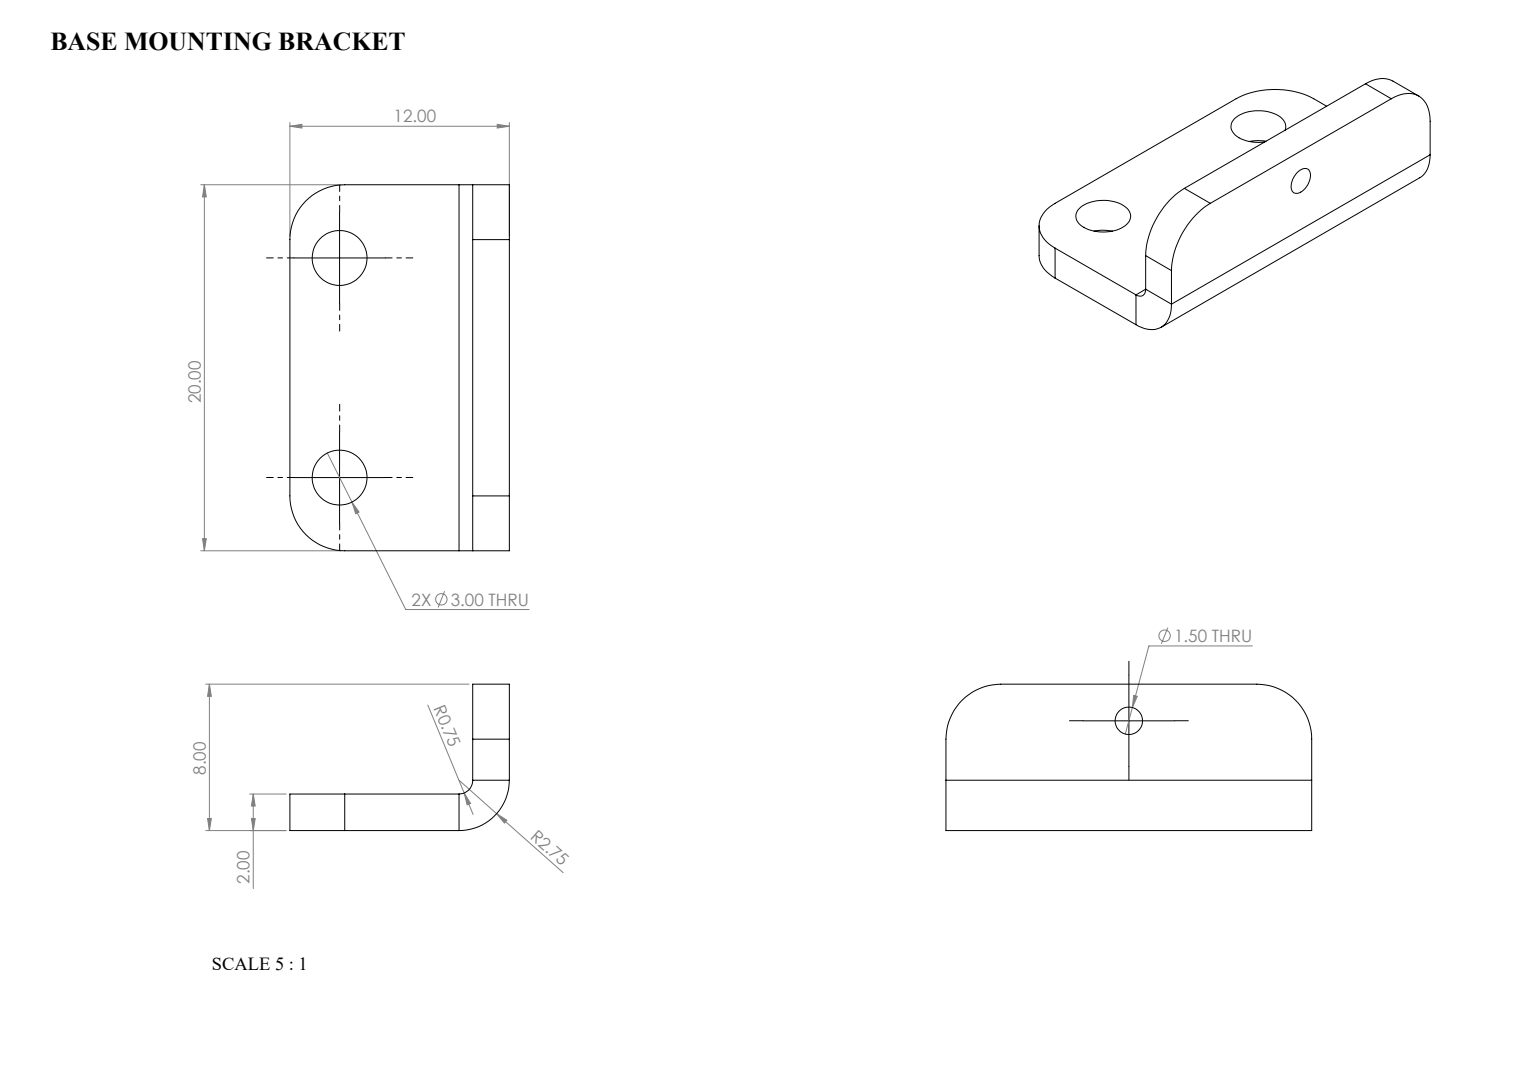
ISO-10303-21;
HEADER;
FILE_DESCRIPTION (('STEP AP214'),
    '1' );
FILE_NAME ('base-mounting-bracket.step',
    '2026-10-11T23:18:24',
    ( '' ),
    ( '' ),
    'SwSTEP 2.0',
    'SolidWorks 2021',
    '' );
FILE_SCHEMA (( 'AUTOMOTIVE_DESIGN' ));
ENDSEC;

DATA;
#8=ORIENTED_EDGE ( 'NONE', *, *, #949, .F. ) ;
#37=FACE_OUTER_BOUND ( 'NONE', #7927, .T. ) ;
#43=VERTEX_POINT ( 'NONE', #6242 ) ;
#47=FACE_BOUND ( 'NONE', #7549, .T. ) ;
#50=CIRCLE ( 'NONE', #7727, 3.000000000000000000 ) ;
#51=FACE_OUTER_BOUND ( 'NONE', #63, .T. ) ;
#63=EDGE_LOOP ( 'NONE', ( #5168, #8136, #3931, #2663 ) ) ;
#72=CARTESIAN_POINT ( 'NONE',  ( 10.00000000000000000, 2.749999999999999112, -10.00000000000000178 ) ) ;
#122=AXIS2_PLACEMENT_3D ( 'NONE', #7328, #11458, #1060 ) ;
#142=FACE_OUTER_BOUND ( 'NONE', #3099, .T. ) ;
#145=ORIENTED_EDGE ( 'NONE', *, *, #11996, .T. ) ;
#170=DIRECTION ( 'NONE',  ( -2.602085213965199795E-16, 2.891205793294684736E-16, -1.000000000000000000 ) ) ;
#212=EDGE_CURVE ( 'NONE', #8880, #8783, #12663, .T. ) ;
#240=ORIENTED_EDGE ( 'NONE', *, *, #11722, .F. ) ;
#241=DIRECTION ( 'NONE',  ( 0.000000000000000000, 1.000000000000000000, -0.000000000000000000 ) ) ;
#257=LINE ( 'NONE', #1752, #8132 ) ;
#264=EDGE_CURVE ( 'NONE', #8710, #692, #9279, .T. ) ;
#268=EDGE_LOOP ( 'NONE', ( #11853, #9948, #1249, #11697 ) ) ;
#271=EDGE_CURVE ( 'NONE', #7435, #2693, #13455, .T. ) ;
#304=DIRECTION ( 'NONE',  ( 0.000000000000000000, 1.000000000000000000, 0.000000000000000000 ) ) ;
#311=CIRCLE ( 'NONE', #11742, 3.000000000000000000 ) ;
#329=CARTESIAN_POINT ( 'NONE',  ( 2.720000000000001528, 2.000000000000000000, 7.500000000000000888 ) ) ;
#374=ORIENTED_EDGE ( 'NONE', *, *, #11346, .F. ) ;
#420=CARTESIAN_POINT ( 'NONE',  ( 2.720000000000001528, 0.000000000000000000, 4.500000000000000000 ) ) ;
#425=ORIENTED_EDGE ( 'NONE', *, *, #11861, .F. ) ;
#444=EDGE_CURVE ( 'NONE', #11209, #5642, #3242, .T. ) ;
#445=MECHANICAL_DESIGN_GEOMETRIC_PRESENTATION_REPRESENTATION('',(#6386),#6171);
#474=LINE ( 'NONE', #4679, #13306 ) ;
#486=ORIENTED_EDGE ( 'NONE', *, *, #11722, .T. ) ;
#489=( NAMED_UNIT ( * ) SI_UNIT ( $, .STERADIAN. ) SOLID_ANGLE_UNIT ( ) );
#491=AXIS2_PLACEMENT_3D ( 'NONE', #848, #12295, #6081 ) ;
#519=VECTOR ( 'NONE', #1899, 1000.000000000000000 ) ;
#559=EDGE_LOOP ( 'NONE', ( #8381, #3710, #2080, #13458 ) ) ;
#563=LINE ( 'NONE', #1798, #9730 ) ;
#590=DIRECTION ( 'NONE',  ( 0.000000000000000000, 0.000000000000000000, 1.000000000000000000 ) ) ;
#599=FACE_OUTER_BOUND ( 'NONE', #1472, .T. ) ;
#603=DIRECTION ( 'NONE',  ( 1.000000000000000000, -3.469446951953610639E-15, -2.602085213965210149E-16 ) ) ;
#608=ORIENTED_EDGE ( 'NONE', *, *, #6998, .F. ) ;
#614=ADVANCED_FACE ( 'NONE', ( #3441 ), #10691, .F. ) ;
#631=DIRECTION ( 'NONE',  ( 0.000000000000000000, 0.000000000000000000, -1.000000000000000000 ) ) ;
#639=ADVANCED_BREP_SHAPE_REPRESENTATION ( '', ( #3911, #10007 ), #12660 ) ;
#648=DIRECTION ( 'NONE',  ( -3.469446951953614189E-15, -1.000000000000000000, 8.673617379884035472E-16 ) ) ;
#687=LINE ( 'NONE', #5850, #12010 ) ;
#692=VERTEX_POINT ( 'NONE', #11854 ) ;
#697=ORIENTED_EDGE ( 'NONE', *, *, #1747, .T. ) ;
#707=EDGE_CURVE ( 'NONE', #8736, #9662, #5546, .T. ) ;
#736=EDGE_CURVE ( 'NONE', #7676, #11515, #12131, .T. ) ;
#740=AXIS2_PLACEMENT_3D ( 'NONE', #5209, #10447, #871 ) ;
#808=ORIENTED_EDGE ( 'NONE', *, *, #12116, .F. ) ;
#810=LINE ( 'NONE', #12316, #2307 ) ;
#848=CARTESIAN_POINT ( 'NONE',  ( 10.00000000000001421, 6.000000000000007105, -2.602085213965208275E-15 ) ) ;
#854=DIRECTION ( 'NONE',  ( -1.000000000000000000, 0.000000000000000000, -0.000000000000000000 ) ) ;
#865=ORIENTED_EDGE ( 'NONE', *, *, #444, .T. ) ;
#871=DIRECTION ( 'NONE',  ( 0.000000000000000000, 0.000000000000000000, 1.000000000000000000 ) ) ;
#872=EDGE_CURVE ( 'NONE', #8783, #8207, #563, .T. ) ;
#901=SURFACE_SIDE_STYLE ('',( #11166 ) ) ;
#940=LINE ( 'NONE', #9342, #5056 ) ;
#949=EDGE_CURVE ( 'NONE', #11231, #5642, #6128, .T. ) ;
#954=DIRECTION ( 'NONE',  ( 0.000000000000000000, 0.000000000000000000, 1.000000000000000000 ) ) ;
#971=DIRECTION ( 'NONE',  ( 0.000000000000000000, 0.000000000000000000, 1.000000000000000000 ) ) ;
#978=ORIENTED_EDGE ( 'NONE', *, *, #10739, .T. ) ;
#994=CARTESIAN_POINT ( 'NONE',  ( 12.00000000000000533, 2.749999999999991118, 10.00000000000000000 ) ) ;
#1001=ORIENTED_EDGE ( 'NONE', *, *, #5458, .F. ) ;
#1060=DIRECTION ( 'NONE',  ( 0.000000000000000000, 0.000000000000000000, 1.000000000000000000 ) ) ;
#1071=DIRECTION ( 'NONE',  ( -2.312964634635743450E-15, -1.000000000000000000, 0.000000000000000000 ) ) ;
#1102=EDGE_CURVE ( 'NONE', #43, #2399, #1440, .T. ) ;
#1136=DIRECTION ( 'NONE',  ( 2.602085213965210149E-16, 0.000000000000000000, 1.000000000000000000 ) ) ;
#1141=DIRECTION ( 'NONE',  ( 0.000000000000000000, 0.000000000000000000, 1.000000000000000000 ) ) ;
#1145=CIRCLE ( 'NONE', #4886, 0.7500000000000024425 ) ;
#1146=CARTESIAN_POINT ( 'NONE',  ( 3.000000000000001776, 2.000000000000000000, 10.00000000000000000 ) ) ;
#1174=CIRCLE ( 'NONE', #740, 1.499999999999999556 ) ;
#1185=ORIENTED_EDGE ( 'NONE', *, *, #10601, .F. ) ;
#1223=CARTESIAN_POINT ( 'NONE',  ( -2.551540321038929007E-15, 0.000000000000000000, -7.000000000000000000 ) ) ;
#1249=ORIENTED_EDGE ( 'NONE', *, *, #3731, .T. ) ;
#1266=VERTEX_POINT ( 'NONE', #11146 ) ;
#1282=ADVANCED_FACE ( 'NONE', ( #1650 ), #6793, .F. ) ;
#1358=EDGE_LOOP ( 'NONE', ( #6259, #10717, #6942, #8787 ) ) ;
#1361=ORIENTED_EDGE ( 'NONE', *, *, #4222, .F. ) ;
#1367=VECTOR ( 'NONE', #2475, 1000.000000000000000 ) ;
#1378=ORIENTED_EDGE ( 'NONE', *, *, #7513, .T. ) ;
#1384=DIRECTION ( 'NONE',  ( 0.000000000000000000, 1.000000000000000000, 0.000000000000000000 ) ) ;
#1395=AXIS2_PLACEMENT_3D ( 'NONE', #11099, #6753, #631 ) ;
#1399=ORIENTED_EDGE ( 'NONE', *, *, #4811, .F. ) ;
#1421=CARTESIAN_POINT ( 'NONE',  ( 9.250000000000001776, 1.999999999999998224, -10.00000000000000178 ) ) ;
#1440=LINE ( 'NONE', #9630, #11953 ) ;
#1459=DIRECTION ( 'NONE',  ( 2.602085213965199795E-16, -2.891205793294684736E-16, 1.000000000000000000 ) ) ;
#1472=EDGE_LOOP ( 'NONE', ( #7725, #6948, #2931, #9761 ) ) ;
#1499=ORIENTED_EDGE ( 'NONE', *, *, #9261, .F. ) ;
#1519=ADVANCED_FACE ( 'NONE', ( #13186 ), #3739, .T. ) ;
#1545=DIRECTION ( 'NONE',  ( 1.000000000000000000, -3.469446951953610639E-15, -2.602085213965210149E-16 ) ) ;
#1586=UNCERTAINTY_MEASURE_WITH_UNIT (LENGTH_MEASURE( 1.000000000000000082E-05 ), #6895, 'distance_accuracy_value', 'NONE');
#1610=ORIENTED_EDGE ( 'NONE', *, *, #1879, .T. ) ;
#1621=CARTESIAN_POINT ( 'NONE',  ( 20.00000000000001421, 5.999999999999972466, -5.204170427930418128E-15 ) ) ;
#1650=FACE_OUTER_BOUND ( 'NONE', #4981, .T. ) ;
#1662=VERTEX_POINT ( 'NONE', #329 ) ;
#1669=CYLINDRICAL_SURFACE ( 'NONE', #1395, 1.500000000000000444 ) ;
#1674=DIRECTION ( 'NONE',  ( -2.312964634635743450E-15, -1.000000000000000000, 0.000000000000000000 ) ) ;
#1697=ORIENTED_EDGE ( 'NONE', *, *, #10199, .F. ) ;
#1723=CARTESIAN_POINT ( 'NONE',  ( 12.00000000000001243, 4.999999999999999112, 10.00000000000000178 ) ) ;
#1732=ADVANCED_FACE ( 'NONE', ( #9746 ), #6375, .F. ) ;
#1740=CARTESIAN_POINT ( 'NONE',  ( 12.00000000000001421, 6.000000000000000000, -3.122502256758250009E-15 ) ) ;
#1747=EDGE_CURVE ( 'NONE', #2399, #7044, #7623, .T. ) ;
#1752=CARTESIAN_POINT ( 'NONE',  ( 11.99999999999999112, -4.572512030783488065E-14, -10.00000000000000178 ) ) ;
#1798=CARTESIAN_POINT ( 'NONE',  ( 3.000000000000001776, 0.000000000000000000, 10.00000000000000000 ) ) ;
#1809=LINE ( 'NONE', #6824, #4723 ) ;
#1862=LINE ( 'NONE', #7167, #5318 ) ;
#1872=ORIENTED_EDGE ( 'NONE', *, *, #3526, .F. ) ;
#1879=EDGE_CURVE ( 'NONE', #2097, #9662, #3747, .T. ) ;
#1888=EDGE_LOOP ( 'NONE', ( #6480, #9877 ) ) ;
#1899=DIRECTION ( 'NONE',  ( 1.000000000000000000, -3.491481338843133355E-15, -2.602085213965210149E-16 ) ) ;
#1913=DIRECTION ( 'NONE',  ( -0.000000000000000000, -1.000000000000000000, -0.000000000000000000 ) ) ;
#1938=FILL_AREA_STYLE_COLOUR ( '', #13317 ) ;
#1950=CARTESIAN_POINT ( 'NONE',  ( 11.99999999999999467, -5.150753189442425446E-14, 10.00000000000000000 ) ) ;
#1951=ORIENTED_EDGE ( 'NONE', *, *, #8465, .F. ) ;
#1964=EDGE_CURVE ( 'NONE', #5535, #13368, #9406, .T. ) ;
#1994=CARTESIAN_POINT ( 'NONE',  ( 2.720000000000001528, 0.000000000000000000, 7.500000000000000888 ) ) ;
#2028=DIRECTION ( 'NONE',  ( -1.000000000000000000, 3.469446951953610639E-15, 2.602085213965210149E-16 ) ) ;
#2080=ORIENTED_EDGE ( 'NONE', *, *, #1964, .F. ) ;
#2092=AXIS2_PLACEMENT_3D ( 'NONE', #6235, #2858, #3957 ) ;
#2094=CIRCLE ( 'NONE', #122, 1.500000000000000444 ) ;
#2097=VERTEX_POINT ( 'NONE', #6037 ) ;
#2109=DIRECTION ( 'NONE',  ( -3.469446951953614189E-15, -1.000000000000000000, 0.000000000000000000 ) ) ;
#2133=EDGE_CURVE ( 'NONE', #13368, #2399, #8219, .T. ) ;
#2140=LINE ( 'NONE', #5238, #4952 ) ;
#2156=DIRECTION ( 'NONE',  ( 0.000000000000000000, 1.000000000000000000, 0.000000000000000000 ) ) ;
#2165=ORIENTED_EDGE ( 'NONE', *, *, #11291, .T. ) ;
#2185=DIRECTION ( 'NONE',  ( -1.000000000000000000, 3.469446951953610639E-15, 2.602085213965210149E-16 ) ) ;
#2204=ADVANCED_FACE ( 'NONE', ( #11813, #47, #9465 ), #11610, .F. ) ;
#2231=EDGE_CURVE ( 'NONE', #9010, #7333, #4707, .T. ) ;
#2250=DIRECTION ( 'NONE',  ( -3.469446951953610639E-15, -1.000000000000000000, 0.000000000000000000 ) ) ;
#2275=ORIENTED_EDGE ( 'NONE', *, *, #8478, .T. ) ;
#2287=ADVANCED_FACE ( 'NONE', ( #11115 ), #5732, .F. ) ;
#2307=VECTOR ( 'NONE', #11268, 1000.000000000000000 ) ;
#2326=DIRECTION ( 'NONE',  ( 0.000000000000000000, 0.000000000000000000, -1.000000000000000000 ) ) ;
#2327=DIRECTION ( 'NONE',  ( 3.469446951953610639E-15, 1.000000000000000000, 2.891205793294675861E-16 ) ) ;
#2344=CARTESIAN_POINT ( 'NONE',  ( 10.00000000000002309, 8.000000000000007105, 7.000000000000001776 ) ) ;
#2365=ADVANCED_FACE ( 'NONE', ( #7127, #10285, #8279 ), #4084, .T. ) ;
#2394=ORIENTED_EDGE ( 'NONE', *, *, #444, .F. ) ;
#2399=VERTEX_POINT ( 'NONE', #10346 ) ;
#2475=DIRECTION ( 'NONE',  ( -1.000000000000000000, 3.491481338843133355E-15, 2.602085213965210149E-16 ) ) ;
#2485=ORIENTED_EDGE ( 'NONE', *, *, #264, .T. ) ;
#2508=CARTESIAN_POINT ( 'NONE',  ( 12.00000000000000888, 5.000000000000000000, -6.999999999999999112 ) ) ;
#2573=DIRECTION ( 'NONE',  ( -0.000000000000000000, -1.000000000000000000, -0.000000000000000000 ) ) ;
#2621=ADVANCED_FACE ( 'NONE', ( #9786 ), #1669, .F. ) ;
#2627=ORIENTED_EDGE ( 'NONE', *, *, #10538, .T. ) ;
#2658=CARTESIAN_POINT ( 'NONE',  ( 3.000000000000001776, 2.000000000000000000, 10.00000000000000000 ) ) ;
#2663=ORIENTED_EDGE ( 'NONE', *, *, #271, .F. ) ;
#2686=( NAMED_UNIT ( * ) SI_UNIT ( $, .STERADIAN. ) SOLID_ANGLE_UNIT ( ) );
#2693=VERTEX_POINT ( 'NONE', #12900 ) ;
#2695=ADVANCED_FACE ( 'NONE', ( #8882 ), #3711, .T. ) ;
#2702=AXIS2_PLACEMENT_3D ( 'NONE', #12467, #3258, #1071 ) ;
#2735=CARTESIAN_POINT ( 'NONE',  ( 10.00000000000001243, 5.000000000000007105, 7.000000000000001776 ) ) ;
#2761=ORIENTED_EDGE ( 'NONE', *, *, #949, .T. ) ;
#2825=EDGE_CURVE ( 'NONE', #5427, #12707, #3934, .T. ) ;
#2847=DIRECTION ( 'NONE',  ( 0.000000000000000000, 1.000000000000000000, 0.000000000000000000 ) ) ;
#2858=DIRECTION ( 'NONE',  ( -0.000000000000000000, -0.000000000000000000, -1.000000000000000000 ) ) ;
#2867=EDGE_CURVE ( 'NONE', #12707, #5427, #12317, .T. ) ;
#2879=DIRECTION ( 'NONE',  ( -1.000000000000000000, 3.469446951953610639E-15, 2.602085213965210149E-16 ) ) ;
#2895=FILL_AREA_STYLE ('',( #1938 ) ) ;
#2896=CARTESIAN_POINT ( 'NONE',  ( 12.00000000000002309, 8.000000000000000000, 7.000000000000000888 ) ) ;
#2929=ORIENTED_EDGE ( 'NONE', *, *, #11861, .T. ) ;
#2931=ORIENTED_EDGE ( 'NONE', *, *, #8943, .F. ) ;
#2947=EDGE_LOOP ( 'NONE', ( #11195, #11654, #6079, #11465 ) ) ;
#2956=PLANE ( 'NONE',  #12210 ) ;
#2957=VECTOR ( 'NONE', #2879, 1000.000000000000000 ) ;
#3056=AXIS2_PLACEMENT_3D ( 'NONE', #10125, #12284, #971 ) ;
#3083=DIRECTION ( 'NONE',  ( -1.000000000000000000, -0.000000000000000000, -1.927470528863118802E-16 ) ) ;
#3099=EDGE_LOOP ( 'NONE', ( #12485, #7712, #865, #8, #13124, #4158 ) ) ;
#3149=FACE_BOUND ( 'NONE', #3474, .T. ) ;
#3184=CARTESIAN_POINT ( 'NONE',  ( 2.719999999999997087, 2.000000000000000000, -6.000000000000000000 ) ) ;
#3191=PLANE ( 'NONE',  #6195 ) ;
#3202=DIRECTION ( 'NONE',  ( 0.000000000000000000, -0.000000000000000000, 1.000000000000000000 ) ) ;
#3204=DIRECTION ( 'NONE',  ( 1.000000000000000000, 0.000000000000000000, -0.000000000000000000 ) ) ;
#3242=LINE ( 'NONE', #1950, #11944 ) ;
#3251=ORIENTED_EDGE ( 'NONE', *, *, #872, .T. ) ;
#3258=DIRECTION ( 'NONE',  ( -1.000000000000000000, 3.469446951953610639E-15, 2.602085213965210149E-16 ) ) ;
#3266=ORIENTED_EDGE ( 'NONE', *, *, #4811, .T. ) ;
#3381=DIRECTION ( 'NONE',  ( 0.000000000000000000, 0.000000000000000000, 1.000000000000000000 ) ) ;
#3435=CARTESIAN_POINT ( 'NONE',  ( 2.999999999999997335, 2.000000000000000000, -7.000000000000001776 ) ) ;
#3441=FACE_OUTER_BOUND ( 'NONE', #4881, .T. ) ;
#3460=EDGE_CURVE ( 'NONE', #9662, #8736, #4395, .T. ) ;
#3465=DIRECTION ( 'NONE',  ( 1.000000000000000000, -3.469446951953610639E-15, 0.000000000000000000 ) ) ;
#3474=EDGE_LOOP ( 'NONE', ( #978, #8024 ) ) ;
#3486=EDGE_LOOP ( 'NONE', ( #1951, #2929, #1610, #4440 ) ) ;
#3504=CARTESIAN_POINT ( 'NONE',  ( 12.00000000000001776, 8.000000000000000000, -10.00000000000000000 ) ) ;
#3506=ORIENTED_EDGE ( 'NONE', *, *, #707, .T. ) ;
#3508=CIRCLE ( 'NONE', #10568, 1.499999999999999556 ) ;
#3526=EDGE_CURVE ( 'NONE', #11231, #9693, #257, .T. ) ;
#3537=ORIENTED_EDGE ( 'NONE', *, *, #736, .T. ) ;
#3582=DIRECTION ( 'NONE',  ( -1.000000000000000000, 3.491481338843133355E-15, 2.602085213965210149E-16 ) ) ;
#3645=UNCERTAINTY_MEASURE_WITH_UNIT (LENGTH_MEASURE( 1.000000000000000082E-05 ), #12139, 'distance_accuracy_value', 'NONE');
#3706=ORIENTED_EDGE ( 'NONE', *, *, #8465, .T. ) ;
#3710=ORIENTED_EDGE ( 'NONE', *, *, #5809, .T. ) ;
#3711=CYLINDRICAL_SURFACE ( 'NONE', #7428, 3.000000000000000000 ) ;
#3727=VECTOR ( 'NONE', #13392, 1000.000000000000000 ) ;
#3731=EDGE_CURVE ( 'NONE', #6099, #8207, #4986, .T. ) ;
#3739=PLANE ( 'NONE',  #6891 ) ;
#3747=LINE ( 'NONE', #13269, #5349 ) ;
#3809=ADVANCED_FACE ( 'NONE', ( #9653 ), #7656, .F. ) ;
#3814=CARTESIAN_POINT ( 'NONE',  ( 2.719999999999997087, 2.000000000000000000, -6.000000000000000000 ) ) ;
#3817=AXIS2_PLACEMENT_3D ( 'NONE', #10664, #10589, #2326 ) ;
#3866=DIRECTION ( 'NONE',  ( -0.000000000000000000, -0.000000000000000000, -1.000000000000000000 ) ) ;
#3880=CARTESIAN_POINT ( 'NONE',  ( 10.00000000000000533, 2.749999999999997335, 10.00000000000000178 ) ) ;
#3911=MANIFOLD_SOLID_BREP ( 'Fillet1', #5975 ) ;
#3925=DIRECTION ( 'NONE',  ( -4.625929269271486900E-15, -1.000000000000000000, 0.000000000000000000 ) ) ;
#3931=ORIENTED_EDGE ( 'NONE', *, *, #13097, .T. ) ;
#3934=CIRCLE ( 'NONE', #3056, 1.499999999999999556 ) ;
#3935=ORIENTED_EDGE ( 'NONE', *, *, #7589, .T. ) ;
#3957=DIRECTION ( 'NONE',  ( -1.000000000000000000, 0.000000000000000000, 0.000000000000000000 ) ) ;
#3984=CARTESIAN_POINT ( 'NONE',  ( 2.999999999999995559, 2.000000000000000000, -10.00000000000000355 ) ) ;
#4040=ADVANCED_FACE ( 'NONE', ( #13378 ), #10272, .F. ) ;
#4052=DIRECTION ( 'NONE',  ( -1.927470528863118802E-16, 0.000000000000000000, 1.000000000000000000 ) ) ;
#4069=CARTESIAN_POINT ( 'NONE',  ( 12.00000000000001599, 6.750000000000000000, -2.770445225425678373E-15 ) ) ;
#4084=PLANE ( 'NONE',  #8441 ) ;
#4099=ORIENTED_EDGE ( 'NONE', *, *, #5220, .T. ) ;
#4158=ORIENTED_EDGE ( 'NONE', *, *, #5458, .T. ) ;
#4168=ORIENTED_EDGE ( 'NONE', *, *, #11566, .F. ) ;
#4196=DIRECTION ( 'NONE',  ( 0.000000000000000000, 0.000000000000000000, -1.000000000000000000 ) ) ;
#4222=EDGE_CURVE ( 'NONE', #8880, #6099, #8464, .T. ) ;
#4230=CARTESIAN_POINT ( 'NONE',  ( 3.000000000000001776, 0.000000000000000000, 7.000000000000000000 ) ) ;
#4232=PLANE ( 'NONE',  #4692 ) ;
#4246=PRODUCT_DEFINITION_SHAPE ( 'NONE', 'NONE',  #5460 ) ;
#4273=DIRECTION ( 'NONE',  ( 1.000000000000000000, -3.469446951953602750E-15, 0.000000000000000000 ) ) ;
#4302=CIRCLE ( 'NONE', #10463, 3.000000000000000000 ) ;
#4317=VERTEX_POINT ( 'NONE', #6875 ) ;
#4331=ORIENTED_EDGE ( 'NONE', *, *, #10538, .F. ) ;
#4375=ORIENTED_EDGE ( 'NONE', *, *, #13136, .T. ) ;
#4390=VERTEX_POINT ( 'NONE', #12196 ) ;
#4395=CIRCLE ( 'NONE', #12763, 1.500000000000000444 ) ;
#4404=APPLICATION_CONTEXT ( 'automotive_design' ) ;
#4417=DIRECTION ( 'NONE',  ( -0.000000000000000000, -1.000000000000000000, -0.000000000000000000 ) ) ;
#4439=CARTESIAN_POINT ( 'NONE',  ( 10.00000000000001243, 5.000000000000006217, 10.00000000000000178 ) ) ;
#4440=ORIENTED_EDGE ( 'NONE', *, *, #707, .F. ) ;
#4534=ORIENTED_EDGE ( 'NONE', *, *, #3731, .F. ) ;
#4535=DIRECTION ( 'NONE',  ( -0.000000000000000000, -1.000000000000000000, -0.000000000000000000 ) ) ;
#4545=CYLINDRICAL_SURFACE ( 'NONE', #7126, 3.000000000000000000 ) ;
#4585=ORIENTED_EDGE ( 'NONE', *, *, #13097, .F. ) ;
#4617=AXIS2_PLACEMENT_3D ( 'NONE', #1621, #5816, #10014 ) ;
#4633=DIRECTION ( 'NONE',  ( 2.602085213965210149E-16, -0.000000000000000000, 1.000000000000000000 ) ) ;
#4657=VECTOR ( 'NONE', #5345, 1000.000000000000000 ) ;
#4679=CARTESIAN_POINT ( 'NONE',  ( 12.00000000000000355, 2.749999999999990230, 10.00000000000000000 ) ) ;
#4692=AXIS2_PLACEMENT_3D ( 'NONE', #8428, #12653, #3204 ) ;
#4703=AXIS2_PLACEMENT_3D ( 'NONE', #7037, #6758, #1674 ) ;
#4707=LINE ( 'NONE', #4778, #10156 ) ;
#4723=VECTOR ( 'NONE', #4771, 1000.000000000000000 ) ;
#4771=DIRECTION ( 'NONE',  ( -0.000000000000000000, -1.000000000000000000, -0.000000000000000000 ) ) ;
#4778=CARTESIAN_POINT ( 'NONE',  ( 10.00000000000002309, 8.000000000000007105, 10.00000000000000178 ) ) ;
#4782=CARTESIAN_POINT ( 'NONE',  ( 2.719999999999997087, 0.000000000000000000, -4.500000000000000888 ) ) ;
#4787=DIRECTION ( 'NONE',  ( 0.000000000000000000, 1.000000000000000000, -0.000000000000000000 ) ) ;
#4793=DIRECTION ( 'NONE',  ( -3.469446951953614189E-15, -1.000000000000000000, 0.000000000000000000 ) ) ;
#4811=EDGE_CURVE ( 'NONE', #9688, #692, #4936, .T. ) ;
#4845=FACE_OUTER_BOUND ( 'NONE', #7120, .T. ) ;
#4881=EDGE_LOOP ( 'NONE', ( #8205, #2627, #1872, #4168 ) ) ;
#4886=AXIS2_PLACEMENT_3D ( 'NONE', #7738, #10917, #11752 ) ;
#4894=CARTESIAN_POINT ( 'NONE',  ( 20.00000000000001421, 5.999999999999972466, -5.204170427930418128E-15 ) ) ;
#4895=AXIS2_PLACEMENT_3D ( 'NONE', #3504, #1459, #9910 ) ;
#4902=CYLINDRICAL_SURFACE ( 'NONE', #11110, 0.7500000000000024425 ) ;
#4910=VECTOR ( 'NONE', #6198, 1000.000000000000000 ) ;
#4936=LINE ( 'NONE', #9055, #10113 ) ;
#4952=VECTOR ( 'NONE', #13448, 1000.000000000000000 ) ;
#4959=CARTESIAN_POINT ( 'NONE',  ( 10.00000000000001243, 5.250000000000007105, -2.602085213965208275E-15 ) ) ;
#4981=EDGE_LOOP ( 'NONE', ( #697, #12186, #7245, #12343 ) ) ;
#4986=LINE ( 'NONE', #9179, #3727 ) ;
#4989=LINE ( 'NONE', #3880, #13457 ) ;
#5020=LINE ( 'NONE', #3984, #6939 ) ;
#5031=EDGE_CURVE ( 'NONE', #4317, #12707, #940, .T. ) ;
#5032=DIRECTION ( 'NONE',  ( -0.000000000000000000, -1.000000000000000000, -0.000000000000000000 ) ) ;
#5056=VECTOR ( 'NONE', #8300, 1000.000000000000000 ) ;
#5057=AXIS2_PLACEMENT_3D ( 'NONE', #9448, #170, #12834 ) ;
#5058=ORIENTED_EDGE ( 'NONE', *, *, #872, .F. ) ;
#5085=CARTESIAN_POINT ( 'NONE',  ( 20.00000000000001066, 5.249999999999972466, -5.204170427930418128E-15 ) ) ;
#5091=ORIENTED_EDGE ( 'NONE', *, *, #12432, .F. ) ;
#5131=ADVANCED_FACE ( 'NONE', ( #9809 ), #9669, .T. ) ;
#5168=ORIENTED_EDGE ( 'NONE', *, *, #7731, .F. ) ;
#5170=CIRCLE ( 'NONE', #7155, 1.500000000000000444 ) ;
#5209=CARTESIAN_POINT ( 'NONE',  ( 2.719999999999997087, 2.000000000000000000, -6.000000000000000000 ) ) ;
#5220=EDGE_CURVE ( 'NONE', #11515, #1266, #4989, .T. ) ;
#5238=CARTESIAN_POINT ( 'NONE',  ( 10.00000000000001954, 8.000000000000007105, -10.00000000000000000 ) ) ;
#5292=ADVANCED_FACE ( 'NONE', ( #4845 ), #12304, .F. ) ;
#5309=EDGE_CURVE ( 'NONE', #6406, #4317, #3508, .T. ) ;
#5318=VECTOR ( 'NONE', #1141, 1000.000000000000000 ) ;
#5324=ORIENTED_EDGE ( 'NONE', *, *, #12397, .T. ) ;
#5329=AXIS2_PLACEMENT_3D ( 'NONE', #10813, #1384, #5580 ) ;
#5345=DIRECTION ( 'NONE',  ( -0.000000000000000000, -1.000000000000000000, -0.000000000000000000 ) ) ;
#5349=VECTOR ( 'NONE', #13192, 1000.000000000000000 ) ;
#5380=CIRCLE ( 'NONE', #9999, 3.000000000000000000 ) ;
#5400=CARTESIAN_POINT ( 'NONE',  ( 2.999999999999997335, 0.000000000000000000, -7.000000000000001776 ) ) ;
#5425=ORIENTED_EDGE ( 'NONE', *, *, #12432, .T. ) ;
#5427=VERTEX_POINT ( 'NONE', #4782 ) ;
#5438=DIRECTION ( 'NONE',  ( -0.000000000000000000, -1.000000000000000000, -0.000000000000000000 ) ) ;
#5458=EDGE_CURVE ( 'NONE', #9693, #9925, #11669, .T. ) ;
#5460=PRODUCT_DEFINITION ( 'UNKNOWN', '', #12680, #7098 ) ;
#5518=CARTESIAN_POINT ( 'NONE',  ( 10.00000000000000888, 5.000000000000007105, -6.999999999999998224 ) ) ;
#5535=VERTEX_POINT ( 'NONE', #8343 ) ;
#5542=ORIENTED_EDGE ( 'NONE', *, *, #7513, .F. ) ;
#5546=CIRCLE ( 'NONE', #5329, 1.500000000000000444 ) ;
#5557=VERTEX_POINT ( 'NONE', #12302 ) ;
#5580=DIRECTION ( 'NONE',  ( 0.000000000000000000, 0.000000000000000000, 1.000000000000000000 ) ) ;
#5585=CARTESIAN_POINT ( 'NONE',  ( 12.00000000000000711, 5.000000000000000000, -6.999999999999999112 ) ) ;
#5596=AXIS2_PLACEMENT_3D ( 'NONE', #12798, #2185, #2250 ) ;
#5635=ADVANCED_FACE ( 'NONE', ( #9180 ), #13394, .F. ) ;
#5642=VERTEX_POINT ( 'NONE', #994 ) ;
#5712=DIRECTION ( 'NONE',  ( 1.000000000000000000, 0.000000000000000000, 0.000000000000000000 ) ) ;
#5724=ORIENTED_EDGE ( 'NONE', *, *, #12506, .T. ) ;
#5732=CYLINDRICAL_SURFACE ( 'NONE', #8006, 1.499999999999999556 ) ;
#5782=ORIENTED_EDGE ( 'NONE', *, *, #11317, .T. ) ;
#5790=CIRCLE ( 'NONE', #9750, 3.000000000000000000 ) ;
#5809=EDGE_CURVE ( 'NONE', #2693, #13368, #7020, .T. ) ;
#5812=AXIS2_PLACEMENT_3D ( 'NONE', #8915, #10090, #4793 ) ;
#5816=DIRECTION ( 'NONE',  ( -1.000000000000000000, 3.469446951953610639E-15, 2.602085213965210149E-16 ) ) ;
#5850=CARTESIAN_POINT ( 'NONE',  ( -2.551540321038929007E-15, 2.000000000000000000, -7.000000000000000000 ) ) ;
#5870=EDGE_LOOP ( 'NONE', ( #11821, #3506 ) ) ;
#5875=ORIENTED_EDGE ( 'NONE', *, *, #1879, .F. ) ;
#5886=DIRECTION ( 'NONE',  ( 0.000000000000000000, 0.000000000000000000, -1.000000000000000000 ) ) ;
#5926=( NAMED_UNIT ( * ) PLANE_ANGLE_UNIT ( ) SI_UNIT ( $, .RADIAN. ) );
#5975=CLOSED_SHELL ( 'NONE', ( #4040, #2621, #13509, #2365, #2204, #11319, #5635, #8536, #1282, #10899, #2287, #1732, #1519, #10229, #5131, #12059, #614, #3809, #11496, #11703, #6756, #5292, #12938, #2695 ) ) ;
#5996=VERTEX_POINT ( 'NONE', #6183 ) ;
#6037=CARTESIAN_POINT ( 'NONE',  ( 2.720000000000001528, 2.000000000000000000, 4.500000000000000000 ) ) ;
#6079=ORIENTED_EDGE ( 'NONE', *, *, #7812, .F. ) ;
#6081=DIRECTION ( 'NONE',  ( -2.312964634635743450E-15, -1.000000000000000000, 0.000000000000000000 ) ) ;
#6099=VERTEX_POINT ( 'NONE', #11830 ) ;
#6128=LINE ( 'NONE', #9493, #7765 ) ;
#6130=DIRECTION ( 'NONE',  ( 0.000000000000000000, 1.000000000000000000, 0.000000000000000000 ) ) ;
#6131=CARTESIAN_POINT ( 'NONE',  ( 12.00000000000000888, 5.000000000000000888, -10.00000000000000000 ) ) ;
#6137=ORIENTED_EDGE ( 'NONE', *, *, #212, .T. ) ;
#6153=DIRECTION ( 'NONE',  ( -3.469446951953610639E-15, -1.000000000000000000, 0.000000000000000000 ) ) ;
#6171=( GEOMETRIC_REPRESENTATION_CONTEXT ( 3 ) GLOBAL_UNCERTAINTY_ASSIGNED_CONTEXT ( ( #1586 ) ) GLOBAL_UNIT_ASSIGNED_CONTEXT ( ( #6895, #9992, #489 ) ) REPRESENTATION_CONTEXT ( 'NONE', 'WORKASPACE' ) );
#6183=CARTESIAN_POINT ( 'NONE',  ( 10.00000000000000888, 5.000000000000007994, -10.00000000000000000 ) ) ;
#6185=AXIS2_PLACEMENT_3D ( 'NONE', #4230, #8425, #3202 ) ;
#6189=DIRECTION ( 'NONE',  ( 0.000000000000000000, 1.000000000000000000, 0.000000000000000000 ) ) ;
#6195=AXIS2_PLACEMENT_3D ( 'NONE', #7261, #12639, #10499 ) ;
#6198=DIRECTION ( 'NONE',  ( 1.000000000000000000, -3.491481338843133355E-15, -2.602085213965210149E-16 ) ) ;
#6235=CARTESIAN_POINT ( 'NONE',  ( 9.250000000000003553, 2.750000000000000888, -10.00000000000000178 ) ) ;
#6240=DIRECTION ( 'NONE',  ( 1.000000000000000000, -3.469446951953610639E-15, -2.602085213965210149E-16 ) ) ;
#6242=CARTESIAN_POINT ( 'NONE',  ( -3.469446951953614189E-15, 2.000000000000000000, -6.999999999999998224 ) ) ;
#6253=CIRCLE ( 'NONE', #2092, 2.750000000000002665 ) ;
#6259=ORIENTED_EDGE ( 'NONE', *, *, #8478, .F. ) ;
#6344=ORIENTED_EDGE ( 'NONE', *, *, #3460, .F. ) ;
#6349=LINE ( 'NONE', #6415, #10461 ) ;
#6375=CYLINDRICAL_SURFACE ( 'NONE', #3817, 1.500000000000000444 ) ;
#6381=CARTESIAN_POINT ( 'NONE',  ( 10.00000000000000533, 2.749999999999998224, 10.00000000000000000 ) ) ;
#6386=STYLED_ITEM('',(#13628),#3911);
#6394=EDGE_CURVE ( 'NONE', #4390, #11209, #50, .T. ) ;
#6406=VERTEX_POINT ( 'NONE', #9470 ) ;
#6415=CARTESIAN_POINT ( 'NONE',  ( 2.719999999999997087, 2.000000000000000000, -4.500000000000000888 ) ) ;
#6440=AXIS2_PLACEMENT_3D ( 'NONE', #11433, #6130, #8263 ) ;
#6451=ORIENTED_EDGE ( 'NONE', *, *, #7406, .T. ) ;
#6480=ORIENTED_EDGE ( 'NONE', *, *, #264, .F. ) ;
#6537=SHAPE_REPRESENTATION ( 'base-mounting-bracket', ( #10007 ), #12660 ) ;
#6594=ORIENTED_EDGE ( 'NONE', *, *, #10199, .T. ) ;
#6635=CARTESIAN_POINT ( 'NONE',  ( 2.999999999999995559, 0.000000000000000000, -10.00000000000000355 ) ) ;
#6681=CARTESIAN_POINT ( 'NONE',  ( 9.250000000000001776, 2.000000000000000000, -10.00000000000000178 ) ) ;
#6684=DIRECTION ( 'NONE',  ( -0.000000000000000000, -1.000000000000000000, -0.000000000000000000 ) ) ;
#6693=DIRECTION ( 'NONE',  ( -3.469446951953614189E-15, -1.000000000000000000, 0.000000000000000000 ) ) ;
#6753=DIRECTION ( 'NONE',  ( -0.000000000000000000, -1.000000000000000000, -0.000000000000000000 ) ) ;
#6754=CARTESIAN_POINT ( 'NONE',  ( 0.000000000000000000, 0.000000000000000000, 0.000000000000000000 ) ) ;
#6756=ADVANCED_FACE ( 'NONE', ( #10355 ), #3191, .F. ) ;
#6758=DIRECTION ( 'NONE',  ( -1.000000000000000000, 3.469446951953610639E-15, 2.602085213965210149E-16 ) ) ;
#6759=DIRECTION ( 'NONE',  ( 0.000000000000000000, 0.000000000000000000, 1.000000000000000000 ) ) ;
#6783=CYLINDRICAL_SURFACE ( 'NONE', #5812, 3.000000000000000000 ) ;
#6793=PLANE ( 'NONE',  #7111 ) ;
#6801=DIRECTION ( 'NONE',  ( 1.000000000000000000, -3.469446951953610639E-15, -2.602085213965210149E-16 ) ) ;
#6824=CARTESIAN_POINT ( 'NONE',  ( 1.734723475976807094E-15, 2.000000000000000000, 7.000000000000000000 ) ) ;
#6846=AXIS2_PLACEMENT_3D ( 'NONE', #12918, #9736, #3465 ) ;
#6875=CARTESIAN_POINT ( 'NONE',  ( 2.719999999999997087, 2.000000000000000000, -7.500000000000000000 ) ) ;
#6877=CARTESIAN_POINT ( 'NONE',  ( 12.00000000000000000, 2.749999999999992006, -10.00000000000000178 ) ) ;
#6891=AXIS2_PLACEMENT_3D ( 'NONE', #7946, #12165, #12306 ) ;
#6895=( LENGTH_UNIT ( ) NAMED_UNIT ( * ) SI_UNIT ( .MILLI., .METRE. ) );
#6939=VECTOR ( 'NONE', #3083, 1000.000000000000000 ) ;
#6942=ORIENTED_EDGE ( 'NONE', *, *, #5031, .T. ) ;
#6948=ORIENTED_EDGE ( 'NONE', *, *, #9769, .F. ) ;
#6973=DIRECTION ( 'NONE',  ( -2.312964634635743450E-15, -1.000000000000000000, 0.000000000000000000 ) ) ;
#6998=EDGE_CURVE ( 'NONE', #9688, #5557, #13242, .T. ) ;
#7000=ORIENTED_EDGE ( 'NONE', *, *, #5220, .F. ) ;
#7020=LINE ( 'NONE', #9973, #11901 ) ;
#7022=DIRECTION ( 'NONE',  ( -1.000000000000000000, -1.156482317317867583E-15, 0.000000000000000000 ) ) ;
#7024=ORIENTED_EDGE ( 'NONE', *, *, #2825, .T. ) ;
#7037=CARTESIAN_POINT ( 'NONE',  ( 12.00000000000001421, 6.000000000000000000, -3.122502256758250009E-15 ) ) ;
#7044=VERTEX_POINT ( 'NONE', #9919 ) ;
#7049=AXIS2_PLACEMENT_3D ( 'NONE', #2508, #1545, #648 ) ;
#7098=PRODUCT_DEFINITION_CONTEXT ( 'detailed design', #4404, 'design' ) ;
#7109=( NAMED_UNIT ( * ) PLANE_ANGLE_UNIT ( ) SI_UNIT ( $, .RADIAN. ) );
#7111=AXIS2_PLACEMENT_3D ( 'NONE', #8043, #12264, #13078 ) ;
#7120=EDGE_LOOP ( 'NONE', ( #1399, #12562, #5782, #2485 ) ) ;
#7126=AXIS2_PLACEMENT_3D ( 'NONE', #3435, #6684, #7646 ) ;
#7127=FACE_BOUND ( 'NONE', #7711, .T. ) ;
#7155=AXIS2_PLACEMENT_3D ( 'NONE', #7602, #304, #6759 ) ;
#7156=ORIENTED_EDGE ( 'NONE', *, *, #5809, .F. ) ;
#7162=MECHANICAL_DESIGN_GEOMETRIC_PRESENTATION_REPRESENTATION('',(#9790),#7372);
#7166=DIRECTION ( 'NONE',  ( -1.000000000000000000, 0.000000000000000000, 0.000000000000000000 ) ) ;
#7167=CARTESIAN_POINT ( 'NONE',  ( 9.249999999999996447, -1.734723475976807094E-15, -10.00000000000000355 ) ) ;
#7200=CARTESIAN_POINT ( 'NONE',  ( 3.000000000000001776, 0.000000000000000000, 7.000000000000000000 ) ) ;
#7245=ORIENTED_EDGE ( 'NONE', *, *, #12397, .F. ) ;
#7261=CARTESIAN_POINT ( 'NONE',  ( 12.00000000000002309, 8.000000000000000000, 10.00000000000000178 ) ) ;
#7263=ORIENTED_EDGE ( 'NONE', *, *, #1747, .F. ) ;
#7293=CARTESIAN_POINT ( 'NONE',  ( 9.250000000000003553, 2.750000000000000888, 10.00000000000000000 ) ) ;
#7312=AXIS2_PLACEMENT_3D ( 'NONE', #12657, #12273, #7022 ) ;
#7328=CARTESIAN_POINT ( 'NONE',  ( 2.720000000000001528, 2.000000000000000000, 6.000000000000000000 ) ) ;
#7333=VERTEX_POINT ( 'NONE', #2344 ) ;
#7336=ORIENTED_EDGE ( 'NONE', *, *, #2231, .F. ) ;
#7338=CARTESIAN_POINT ( 'NONE',  ( 2.999999999999995559, 2.000000000000000000, -10.00000000000000355 ) ) ;
#7356=CARTESIAN_POINT ( 'NONE',  ( 2.720000000000001528, 0.000000000000000000, 6.000000000000000000 ) ) ;
#7361=PLANE ( 'NONE',  #5596 ) ;
#7372=( GEOMETRIC_REPRESENTATION_CONTEXT ( 3 ) GLOBAL_UNCERTAINTY_ASSIGNED_CONTEXT ( ( #3645 ) ) GLOBAL_UNIT_ASSIGNED_CONTEXT ( ( #12139, #7109, #2686 ) ) REPRESENTATION_CONTEXT ( 'NONE', 'WORKASPACE' ) );
#7405=EDGE_LOOP ( 'NONE', ( #5542, #4585, #2761, #374 ) ) ;
#7406=EDGE_CURVE ( 'NONE', #11209, #7676, #10946, .T. ) ;
#7414=EDGE_LOOP ( 'NONE', ( #1001, #4331, #9440, #11003 ) ) ;
#7428=AXIS2_PLACEMENT_3D ( 'NONE', #5585, #3582, #6693 ) ;
#7429=CARTESIAN_POINT ( 'NONE',  ( 3.000000000000001776, 0.000000000000000000, 10.00000000000000000 ) ) ;
#7435=VERTEX_POINT ( 'NONE', #6681 ) ;
#7445=ORIENTED_EDGE ( 'NONE', *, *, #8943, .T. ) ;
#7513=EDGE_CURVE ( 'NONE', #2693, #8207, #1862, .T. ) ;
#7538=CIRCLE ( 'NONE', #8623, 3.000000000000000000 ) ;
#7549=EDGE_LOOP ( 'NONE', ( #9086, #7024 ) ) ;
#7582=ORIENTED_EDGE ( 'NONE', *, *, #5309, .F. ) ;
#7589=EDGE_CURVE ( 'NONE', #6099, #11515, #13252, .T. ) ;
#7602=CARTESIAN_POINT ( 'NONE',  ( 2.720000000000001528, 2.000000000000000000, 6.000000000000000000 ) ) ;
#7623=LINE ( 'NONE', #1223, #11522 ) ;
#7646=DIRECTION ( 'NONE',  ( 0.000000000000000000, 0.000000000000000000, -1.000000000000000000 ) ) ;
#7656=PLANE ( 'NONE',  #5057 ) ;
#7676=VERTEX_POINT ( 'NONE', #4439 ) ;
#7706=AXIS2_PLACEMENT_3D ( 'NONE', #4894, #13443, #3925 ) ;
#7711=EDGE_LOOP ( 'NONE', ( #1697, #7582 ) ) ;
#7712=ORIENTED_EDGE ( 'NONE', *, *, #6394, .T. ) ;
#7725=ORIENTED_EDGE ( 'NONE', *, *, #6394, .F. ) ;
#7727=AXIS2_PLACEMENT_3D ( 'NONE', #8301, #6240, #2109 ) ;
#7731=EDGE_CURVE ( 'NONE', #1266, #7435, #1145, .T. ) ;
#7738=CARTESIAN_POINT ( 'NONE',  ( 9.250000000000003553, 2.750000000000000888, -10.00000000000000178 ) ) ;
#7765=VECTOR ( 'NONE', #11500, 1000.000000000000000 ) ;
#7794=DIRECTION ( 'NONE',  ( -3.469446951953614189E-15, -1.000000000000000000, 0.000000000000000000 ) ) ;
#7812=EDGE_CURVE ( 'NONE', #5535, #43, #7538, .T. ) ;
#7826=DIRECTION ( 'NONE',  ( -1.000000000000000000, 3.469446951953610639E-15, 2.602085213965210149E-16 ) ) ;
#7834=DIRECTION ( 'NONE',  ( 1.000000000000000000, 0.000000000000000000, 0.000000000000000000 ) ) ;
#7845=DIRECTION ( 'NONE',  ( -3.469446951953610639E-15, -1.000000000000000000, -2.891205793294675861E-16 ) ) ;
#7927=EDGE_LOOP ( 'NONE', ( #8469, #7445, #7336, #9404, #808, #7000 ) ) ;
#7946=CARTESIAN_POINT ( 'NONE',  ( 9.250000000000003553, 2.750000000000000888, 10.00000000000000000 ) ) ;
#7987=DIRECTION ( 'NONE',  ( 1.000000000000000000, 0.000000000000000000, 0.000000000000000000 ) ) ;
#8001=CARTESIAN_POINT ( 'NONE',  ( 9.250000000000001776, 0.000000000000000000, 10.00000000000000000 ) ) ;
#8005=DIRECTION ( 'NONE',  ( -2.312964634635735561E-15, -1.000000000000000000, 0.000000000000000000 ) ) ;
#8006=AXIS2_PLACEMENT_3D ( 'NONE', #11039, #2573, #8009 ) ;
#8009=DIRECTION ( 'NONE',  ( 0.000000000000000000, 0.000000000000000000, -1.000000000000000000 ) ) ;
#8024=ORIENTED_EDGE ( 'NONE', *, *, #6998, .T. ) ;
#8034=FACE_BOUND ( 'NONE', #1888, .T. ) ;
#8043=CARTESIAN_POINT ( 'NONE',  ( -2.551540321038929007E-15, 2.000000000000000000, -7.000000000000000000 ) ) ;
#8099=DIRECTION ( 'NONE',  ( -1.000000000000000000, 3.469446951953610639E-15, 2.602085213965210149E-16 ) ) ;
#8126=EDGE_LOOP ( 'NONE', ( #12939, #3935, #4099, #13355 ) ) ;
#8132=VECTOR ( 'NONE', #2327, 1000.000000000000000 ) ;
#8136=ORIENTED_EDGE ( 'NONE', *, *, #11566, .T. ) ;
#8144=CARTESIAN_POINT ( 'NONE',  ( 3.000000000000001776, 2.000000000000000000, 10.00000000000000000 ) ) ;
#8205=ORIENTED_EDGE ( 'NONE', *, *, #12116, .T. ) ;
#8207=VERTEX_POINT ( 'NONE', #8001 ) ;
#8211=DIRECTION ( 'NONE',  ( 0.000000000000000000, 1.000000000000000000, 0.000000000000000000 ) ) ;
#8219=CIRCLE ( 'NONE', #11747, 3.000000000000000000 ) ;
#8229=CIRCLE ( 'NONE', #11989, 2.750000000000002665 ) ;
#8263=DIRECTION ( 'NONE',  ( 0.000000000000000000, 0.000000000000000000, 1.000000000000000000 ) ) ;
#8279=FACE_OUTER_BOUND ( 'NONE', #9743, .T. ) ;
#8300=DIRECTION ( 'NONE',  ( -0.000000000000000000, -1.000000000000000000, -0.000000000000000000 ) ) ;
#8301=CARTESIAN_POINT ( 'NONE',  ( 12.00000000000001243, 5.000000000000000000, 7.000000000000000888 ) ) ;
#8313=LINE ( 'NONE', #5085, #2957 ) ;
#8332=EDGE_LOOP ( 'NONE', ( #608, #3266, #13100, #12879 ) ) ;
#8338=DIRECTION ( 'NONE',  ( -0.000000000000000000, -1.000000000000000000, -0.000000000000000000 ) ) ;
#8343=CARTESIAN_POINT ( 'NONE',  ( 2.999999999999995559, 2.000000000000000000, -10.00000000000000355 ) ) ;
#8377=FACE_OUTER_BOUND ( 'NONE', #559, .T. ) ;
#8381=ORIENTED_EDGE ( 'NONE', *, *, #271, .T. ) ;
#8401=DIRECTION ( 'NONE',  ( -3.469446951953610639E-15, -1.000000000000000000, -2.891205793294675861E-16 ) ) ;
#8425=DIRECTION ( 'NONE',  ( 0.000000000000000000, 1.000000000000000000, 0.000000000000000000 ) ) ;
#8428=CARTESIAN_POINT ( 'NONE',  ( 9.250000000000003553, 2.750000000000000888, -10.00000000000000178 ) ) ;
#8441=AXIS2_PLACEMENT_3D ( 'NONE', #12507, #8211, #11179 ) ;
#8464=LINE ( 'NONE', #12688, #12775 ) ;
#8465=EDGE_CURVE ( 'NONE', #1662, #8736, #12819, .T. ) ;
#8469=ORIENTED_EDGE ( 'NONE', *, *, #736, .F. ) ;
#8478=EDGE_CURVE ( 'NONE', #6406, #5427, #6349, .T. ) ;
#8536=ADVANCED_FACE ( 'NONE', ( #12891 ), #4545, .T. ) ;
#8541=DIRECTION ( 'NONE',  ( 0.000000000000000000, 0.000000000000000000, -1.000000000000000000 ) ) ;
#8599=EDGE_LOOP ( 'NONE', ( #11904, #11540, #12263, #4375 ) ) ;
#8623=AXIS2_PLACEMENT_3D ( 'NONE', #12381, #4787, #5886 ) ;
#8632=CIRCLE ( 'NONE', #2702, 0.7499999999999997780 ) ;
#8710=VERTEX_POINT ( 'NONE', #4959 ) ;
#8736=VERTEX_POINT ( 'NONE', #1994 ) ;
#8783=VERTEX_POINT ( 'NONE', #7429 ) ;
#8787=ORIENTED_EDGE ( 'NONE', *, *, #2825, .F. ) ;
#8831=VECTOR ( 'NONE', #7845, 1000.000000000000000 ) ;
#8880=VERTEX_POINT ( 'NONE', #2658 ) ;
#8882=FACE_OUTER_BOUND ( 'NONE', #7414, .T. ) ;
#8915=CARTESIAN_POINT ( 'NONE',  ( 12.00000000000001243, 5.000000000000000000, 7.000000000000000888 ) ) ;
#8943=EDGE_CURVE ( 'NONE', #7676, #7333, #5790, .T. ) ;
#8956=ORIENTED_EDGE ( 'NONE', *, *, #4222, .T. ) ;
#9006=ORIENTED_EDGE ( 'NONE', *, *, #2867, .F. ) ;
#9009=CARTESIAN_POINT ( 'NONE',  ( 10.00000000000000178, 2.000000000000000000, 10.00000000000000000 ) ) ;
#9010=VERTEX_POINT ( 'NONE', #11278 ) ;
#9055=CARTESIAN_POINT ( 'NONE',  ( 20.00000000000001776, 6.749999999999972466, -5.112321917994366767E-15 ) ) ;
#9075=DIRECTION ( 'NONE',  ( 3.061616997868383141E-16, 0.000000000000000000, 1.000000000000000000 ) ) ;
#9086=ORIENTED_EDGE ( 'NONE', *, *, #2867, .T. ) ;
#9120=DIRECTION ( 'NONE',  ( -2.602085213965207190E-16, 8.673617379884034239E-17, -1.000000000000000000 ) ) ;
#9166=CARTESIAN_POINT ( 'NONE',  ( 3.000000000000001776, 2.000000000000000000, 7.000000000000000000 ) ) ;
#9178=DIRECTION ( 'NONE',  ( 0.000000000000000000, 0.000000000000000000, 1.000000000000000000 ) ) ;
#9179=CARTESIAN_POINT ( 'NONE',  ( 9.250000000000001776, 1.999999999999998224, 10.00000000000000000 ) ) ;
#9180=FACE_OUTER_BOUND ( 'NONE', #13002, .T. ) ;
#9225=SURFACE_STYLE_USAGE ( .BOTH. , #901 ) ;
#9227=CYLINDRICAL_SURFACE ( 'NONE', #13061, 3.000000000000000000 ) ;
#9261=EDGE_CURVE ( 'NONE', #7435, #6099, #12634, .T. ) ;
#9279=CIRCLE ( 'NONE', #491, 0.7499999999999997780 ) ;
#9291=UNCERTAINTY_MEASURE_WITH_UNIT (LENGTH_MEASURE( 1.000000000000000082E-05 ), #11929, 'distance_accuracy_value', 'NONE');
#9302=FACE_OUTER_BOUND ( 'NONE', #12664, .T. ) ;
#9336=VERTEX_POINT ( 'NONE', #10425 ) ;
#9342=CARTESIAN_POINT ( 'NONE',  ( 2.719999999999997087, 2.000000000000000000, -7.500000000000000000 ) ) ;
#9395=DIRECTION ( 'NONE',  ( 0.000000000000000000, 0.000000000000000000, 1.000000000000000000 ) ) ;
#9404=ORIENTED_EDGE ( 'NONE', *, *, #11841, .T. ) ;
#9406=LINE ( 'NONE', #7338, #11740 ) ;
#9421=CARTESIAN_POINT ( 'NONE',  ( 2.999999999999995559, 2.000000000000000000, -10.00000000000000355 ) ) ;
#9440=ORIENTED_EDGE ( 'NONE', *, *, #11841, .F. ) ;
#9448=CARTESIAN_POINT ( 'NONE',  ( 12.00000000000000178, 1.999999999999993117, 10.00000000000000000 ) ) ;
#9465=FACE_OUTER_BOUND ( 'NONE', #10435, .T. ) ;
#9470=CARTESIAN_POINT ( 'NONE',  ( 2.719999999999997087, 2.000000000000000000, -4.500000000000000888 ) ) ;
#9493=CARTESIAN_POINT ( 'NONE',  ( 12.00000000000000533, 2.749999999999990230, 10.00000000000000178 ) ) ;
#9526=CARTESIAN_POINT ( 'NONE',  ( 12.00000000000000711, 5.000000000000000888, -10.00000000000000000 ) ) ;
#9555=VECTOR ( 'NONE', #603, 1000.000000000000000 ) ;
#9564=AXIS2_PLACEMENT_3D ( 'NONE', #10500, #2028, #6153 ) ;
#9590=FACE_OUTER_BOUND ( 'NONE', #11303, .T. ) ;
#9630=CARTESIAN_POINT ( 'NONE',  ( -3.469446951953614189E-15, 2.000000000000000000, -6.999999999999998224 ) ) ;
#9651=CYLINDRICAL_SURFACE ( 'NONE', #12462, 1.499999999999999556 ) ;
#9653=FACE_OUTER_BOUND ( 'NONE', #10835, .T. ) ;
#9662=VERTEX_POINT ( 'NONE', #420 ) ;
#9669=CYLINDRICAL_SURFACE ( 'NONE', #6846, 2.750000000000002665 ) ;
#9688=VERTEX_POINT ( 'NONE', #4069 ) ;
#9693=VERTEX_POINT ( 'NONE', #6131 ) ;
#9696=ORIENTED_EDGE ( 'NONE', *, *, #212, .F. ) ;
#9730=VECTOR ( 'NONE', #7987, 1000.000000000000000 ) ;
#9736=DIRECTION ( 'NONE',  ( -0.000000000000000000, -0.000000000000000000, -1.000000000000000000 ) ) ;
#9743=EDGE_LOOP ( 'NONE', ( #8956, #1499, #5724, #12403, #5324, #5425 ) ) ;
#9746=FACE_OUTER_BOUND ( 'NONE', #3486, .T. ) ;
#9750=AXIS2_PLACEMENT_3D ( 'NONE', #2735, #7826, #12044 ) ;
#9761=ORIENTED_EDGE ( 'NONE', *, *, #7406, .F. ) ;
#9769=EDGE_CURVE ( 'NONE', #7333, #4390, #12493, .T. ) ;
#9786=FACE_OUTER_BOUND ( 'NONE', #13221, .T. ) ;
#9790=STYLED_ITEM ( 'NONE', ( #11100 ), #639 ) ;
#9809=FACE_OUTER_BOUND ( 'NONE', #7405, .T. ) ;
#9817=DIRECTION ( 'NONE',  ( 3.061616997868383141E-16, 0.000000000000000000, 1.000000000000000000 ) ) ;
#9823=CARTESIAN_POINT ( 'NONE',  ( 2.719999999999997087, 0.000000000000000000, -7.500000000000000000 ) ) ;
#9877=ORIENTED_EDGE ( 'NONE', *, *, #10073, .F. ) ;
#9910=DIRECTION ( 'NONE',  ( 0.000000000000000000, -1.000000000000000000, -2.891205793294684736E-16 ) ) ;
#9919=CARTESIAN_POINT ( 'NONE',  ( 1.734723475976807094E-15, 0.000000000000000000, 7.000000000000000000 ) ) ;
#9925=VERTEX_POINT ( 'NONE', #13194 ) ;
#9948=ORIENTED_EDGE ( 'NONE', *, *, #7589, .F. ) ;
#9973=CARTESIAN_POINT ( 'NONE',  ( 2.999999999999995559, 0.000000000000000000, -10.00000000000000355 ) ) ;
#9992=( NAMED_UNIT ( * ) PLANE_ANGLE_UNIT ( ) SI_UNIT ( $, .RADIAN. ) );
#9999=AXIS2_PLACEMENT_3D ( 'NONE', #5518, #10902, #7794 ) ;
#10007=AXIS2_PLACEMENT_3D ( 'NONE', #6754, #3381, #5712 ) ;
#10014=DIRECTION ( 'NONE',  ( -4.625929269271486900E-15, -1.000000000000000000, 0.000000000000000000 ) ) ;
#10073=EDGE_CURVE ( 'NONE', #692, #8710, #8632, .T. ) ;
#10090=DIRECTION ( 'NONE',  ( -1.000000000000000000, 3.491481338843133355E-15, 2.602085213965210149E-16 ) ) ;
#10113=VECTOR ( 'NONE', #8099, 1000.000000000000000 ) ;
#10114=APPLICATION_CONTEXT ( 'automotive_design' ) ;
#10125=CARTESIAN_POINT ( 'NONE',  ( 2.719999999999997087, 0.000000000000000000, -6.000000000000000000 ) ) ;
#10131=FACE_OUTER_BOUND ( 'NONE', #8126, .T. ) ;
#10156=VECTOR ( 'NONE', #4633, 1000.000000000000000 ) ;
#10199=EDGE_CURVE ( 'NONE', #4317, #6406, #1174, .T. ) ;
#10229=ADVANCED_FACE ( 'NONE', ( #51 ), #4232, .F. ) ;
#10270=SHAPE_REPRESENTATION_RELATIONSHIP ( 'NONE' , 'NONE' ,  #6537, #639 ) ;
#10272=CYLINDRICAL_SURFACE ( 'NONE', #7706, 0.7499999999999997780 ) ;
#10285=FACE_BOUND ( 'NONE', #13025, .T. ) ;
#10290=DIRECTION ( 'NONE',  ( 0.000000000000000000, 0.000000000000000000, -1.000000000000000000 ) ) ;
#10346=CARTESIAN_POINT ( 'NONE',  ( -3.469446951953614189E-15, 0.000000000000000000, -6.999999999999998224 ) ) ;
#10355=FACE_OUTER_BOUND ( 'NONE', #8599, .T. ) ;
#10390=DIRECTION ( 'NONE',  ( 1.000000000000000000, 0.000000000000000000, 1.927470528863118802E-16 ) ) ;
#10425=CARTESIAN_POINT ( 'NONE',  ( 1.734723475976807094E-15, 2.000000000000000000, 7.000000000000000000 ) ) ;
#10435=EDGE_LOOP ( 'NONE', ( #1378, #5058, #1185, #7263, #10855, #7156 ) ) ;
#10447=DIRECTION ( 'NONE',  ( 0.000000000000000000, 1.000000000000000000, 0.000000000000000000 ) ) ;
#10461=VECTOR ( 'NONE', #8338, 1000.000000000000000 ) ;
#10463=AXIS2_PLACEMENT_3D ( 'NONE', #11295, #6189, #13366 ) ;
#10484=ORIENTED_EDGE ( 'NONE', *, *, #10601, .T. ) ;
#10499=DIRECTION ( 'NONE',  ( 1.000000000000000000, -3.491481338843133355E-15, 0.000000000000000000 ) ) ;
#10500=CARTESIAN_POINT ( 'NONE',  ( 9.999999999999992895, -4.163336342344330085E-14, -2.602085213965208275E-15 ) ) ;
#10538=EDGE_CURVE ( 'NONE', #5996, #9693, #11601, .T. ) ;
#10568=AXIS2_PLACEMENT_3D ( 'NONE', #3814, #2847, #590 ) ;
#10573=CARTESIAN_POINT ( 'NONE',  ( 12.00000000000002132, 8.000000000000000000, -3.122502256758258292E-15 ) ) ;
#10589=DIRECTION ( 'NONE',  ( -0.000000000000000000, -1.000000000000000000, -0.000000000000000000 ) ) ;
#10601=EDGE_CURVE ( 'NONE', #7044, #8783, #311, .T. ) ;
#10631=VECTOR ( 'NONE', #5438, 1000.000000000000000 ) ;
#10664=CARTESIAN_POINT ( 'NONE',  ( 2.720000000000001528, 2.000000000000000000, 6.000000000000000000 ) ) ;
#10691=PLANE ( 'NONE',  #4895 ) ;
#10717=ORIENTED_EDGE ( 'NONE', *, *, #5309, .T. ) ;
#10739=EDGE_CURVE ( 'NONE', #5557, #9688, #11536, .T. ) ;
#10808=CARTESIAN_POINT ( 'NONE',  ( 2.720000000000001528, 2.000000000000000000, 7.500000000000000888 ) ) ;
#10813=CARTESIAN_POINT ( 'NONE',  ( 2.720000000000001528, 0.000000000000000000, 6.000000000000000000 ) ) ;
#10835=EDGE_LOOP ( 'NONE', ( #2394, #6451, #3537, #2165 ) ) ;
#10855=ORIENTED_EDGE ( 'NONE', *, *, #2133, .F. ) ;
#10899=ADVANCED_FACE ( 'NONE', ( #9302 ), #9227, .T. ) ;
#10902=DIRECTION ( 'NONE',  ( -1.000000000000000000, 3.469446951953610639E-15, 2.602085213965210149E-16 ) ) ;
#10917=DIRECTION ( 'NONE',  ( -0.000000000000000000, -0.000000000000000000, -1.000000000000000000 ) ) ;
#10946=LINE ( 'NONE', #12124, #1367 ) ;
#11003=ORIENTED_EDGE ( 'NONE', *, *, #13136, .F. ) ;
#11035=ORIENTED_EDGE ( 'NONE', *, *, #5031, .F. ) ;
#11039=CARTESIAN_POINT ( 'NONE',  ( 2.719999999999997087, 2.000000000000000000, -6.000000000000000000 ) ) ;
#11099=CARTESIAN_POINT ( 'NONE',  ( 2.720000000000001528, 2.000000000000000000, 6.000000000000000000 ) ) ;
#11100=PRESENTATION_STYLE_ASSIGNMENT (( #9225 ) ) ;
#11110=AXIS2_PLACEMENT_3D ( 'NONE', #13315, #3866, #4273 ) ;
#11115=FACE_OUTER_BOUND ( 'NONE', #1358, .T. ) ;
#11146=CARTESIAN_POINT ( 'NONE',  ( 10.00000000000000533, 2.749999999999998224, -10.00000000000000178 ) ) ;
#11166=SURFACE_STYLE_FILL_AREA ( #2895 ) ;
#11179=DIRECTION ( 'NONE',  ( 0.000000000000000000, -0.000000000000000000, 1.000000000000000000 ) ) ;
#11195=ORIENTED_EDGE ( 'NONE', *, *, #2133, .T. ) ;
#11209=VERTEX_POINT ( 'NONE', #1723 ) ;
#11222=AXIS2_PLACEMENT_3D ( 'NONE', #8144, #10290, #854 ) ;
#11231=VERTEX_POINT ( 'NONE', #6877 ) ;
#11268=DIRECTION ( 'NONE',  ( -1.000000000000000000, 3.491481338843133355E-15, 2.602085213965210149E-16 ) ) ;
#11278=CARTESIAN_POINT ( 'NONE',  ( 10.00000000000001776, 8.000000000000007105, -6.999999999999999112 ) ) ;
#11291=EDGE_CURVE ( 'NONE', #11515, #5642, #474, .T. ) ;
#11295=CARTESIAN_POINT ( 'NONE',  ( 3.000000000000001776, 2.000000000000000000, 7.000000000000000000 ) ) ;
#11303=EDGE_LOOP ( 'NONE', ( #6594, #2275, #9006, #11035 ) ) ;
#11317=EDGE_CURVE ( 'NONE', #5557, #8710, #8313, .T. ) ;
#11319=ADVANCED_FACE ( 'NONE', ( #8377 ), #2956, .F. ) ;
#11346=EDGE_CURVE ( 'NONE', #8207, #5642, #8229, .T. ) ;
#11422=SHAPE_DEFINITION_REPRESENTATION ( #4246, #6537 ) ;
#11433=CARTESIAN_POINT ( 'NONE',  ( 2.719999999999997087, 0.000000000000000000, -6.000000000000000000 ) ) ;
#11458=DIRECTION ( 'NONE',  ( 0.000000000000000000, 1.000000000000000000, 0.000000000000000000 ) ) ;
#11465=ORIENTED_EDGE ( 'NONE', *, *, #1964, .T. ) ;
#11496=ADVANCED_FACE ( 'NONE', ( #3149, #142 ), #7361, .F. ) ;
#11500=DIRECTION ( 'NONE',  ( 2.602085213965207190E-16, -8.673617379884034239E-17, 1.000000000000000000 ) ) ;
#11515=VERTEX_POINT ( 'NONE', #6381 ) ;
#11522=VECTOR ( 'NONE', #9817, 1000.000000000000000 ) ;
#11536=CIRCLE ( 'NONE', #4703, 0.7499999999999997780 ) ;
#11540=ORIENTED_EDGE ( 'NONE', *, *, #9769, .T. ) ;
#11544=VECTOR ( 'NONE', #1136, 1000.000000000000000 ) ;
#11566=EDGE_CURVE ( 'NONE', #1266, #11231, #12672, .T. ) ;
#11601=LINE ( 'NONE', #9526, #519 ) ;
#11610=PLANE ( 'NONE',  #6185 ) ;
#11654=ORIENTED_EDGE ( 'NONE', *, *, #1102, .F. ) ;
#11669=CIRCLE ( 'NONE', #7049, 3.000000000000000000 ) ;
#11697=ORIENTED_EDGE ( 'NONE', *, *, #11346, .T. ) ;
#11703=ADVANCED_FACE ( 'NONE', ( #8034, #37 ), #12706, .T. ) ;
#11716=VECTOR ( 'NONE', #9178, 1000.000000000000000 ) ;
#11722=EDGE_CURVE ( 'NONE', #2097, #1662, #2094, .T. ) ;
#11740=VECTOR ( 'NONE', #1913, 1000.000000000000000 ) ;
#11742=AXIS2_PLACEMENT_3D ( 'NONE', #7200, #2156, #9395 ) ;
#11747=AXIS2_PLACEMENT_3D ( 'NONE', #5400, #241, #12914 ) ;
#11752=DIRECTION ( 'NONE',  ( -1.000000000000000000, 0.000000000000000000, 0.000000000000000000 ) ) ;
#11813=FACE_BOUND ( 'NONE', #5870, .T. ) ;
#11821=ORIENTED_EDGE ( 'NONE', *, *, #3460, .T. ) ;
#11830=CARTESIAN_POINT ( 'NONE',  ( 9.250000000000001776, 2.000000000000000000, 10.00000000000000000 ) ) ;
#11841=EDGE_CURVE ( 'NONE', #9010, #5996, #5380, .T. ) ;
#11853=ORIENTED_EDGE ( 'NONE', *, *, #11291, .F. ) ;
#11854=CARTESIAN_POINT ( 'NONE',  ( 10.00000000000001599, 6.750000000000007105, -2.770445225425678767E-15 ) ) ;
#11861=EDGE_CURVE ( 'NONE', #1662, #2097, #5170, .T. ) ;
#11901=VECTOR ( 'NONE', #12336, 1000.000000000000000 ) ;
#11904=ORIENTED_EDGE ( 'NONE', *, *, #2231, .T. ) ;
#11929=( LENGTH_UNIT ( ) NAMED_UNIT ( * ) SI_UNIT ( .MILLI., .METRE. ) );
#11944=VECTOR ( 'NONE', #8401, 1000.000000000000000 ) ;
#11953=VECTOR ( 'NONE', #4535, 1000.000000000000000 ) ;
#11989=AXIS2_PLACEMENT_3D ( 'NONE', #7293, #12603, #7166 ) ;
#11996=EDGE_CURVE ( 'NONE', #9336, #7044, #1809, .T. ) ;
#12010=VECTOR ( 'NONE', #9075, 1000.000000000000000 ) ;
#12044=DIRECTION ( 'NONE',  ( -3.469446951953614189E-15, -1.000000000000000000, 0.000000000000000000 ) ) ;
#12059=ADVANCED_FACE ( 'NONE', ( #10131 ), #4902, .F. ) ;
#12116=EDGE_CURVE ( 'NONE', #1266, #5996, #2140, .T. ) ;
#12124=CARTESIAN_POINT ( 'NONE',  ( 12.00000000000001243, 4.999999999999999112, 10.00000000000000178 ) ) ;
#12131=LINE ( 'NONE', #9009, #8831 ) ;
#12139=( LENGTH_UNIT ( ) NAMED_UNIT ( * ) SI_UNIT ( .MILLI., .METRE. ) );
#12165=DIRECTION ( 'NONE',  ( 0.000000000000000000, 0.000000000000000000, 1.000000000000000000 ) ) ;
#12186=ORIENTED_EDGE ( 'NONE', *, *, #11996, .F. ) ;
#12196=CARTESIAN_POINT ( 'NONE',  ( 12.00000000000002309, 8.000000000000000000, 7.000000000000000888 ) ) ;
#12210=AXIS2_PLACEMENT_3D ( 'NONE', #9421, #4052, #10390 ) ;
#12263=ORIENTED_EDGE ( 'NONE', *, *, #13235, .F. ) ;
#12264=DIRECTION ( 'NONE',  ( 1.000000000000000000, 0.000000000000000000, -3.061616997868383141E-16 ) ) ;
#12273=DIRECTION ( 'NONE',  ( 0.000000000000000000, 0.000000000000000000, 1.000000000000000000 ) ) ;
#12284=DIRECTION ( 'NONE',  ( 0.000000000000000000, 1.000000000000000000, 0.000000000000000000 ) ) ;
#12295=DIRECTION ( 'NONE',  ( -1.000000000000000000, 3.469446951953610639E-15, 2.602085213965210149E-16 ) ) ;
#12302=CARTESIAN_POINT ( 'NONE',  ( 12.00000000000001243, 5.250000000000000000, -3.122502256758250009E-15 ) ) ;
#12304=CYLINDRICAL_SURFACE ( 'NONE', #4617, 0.7499999999999997780 ) ;
#12306=DIRECTION ( 'NONE',  ( 1.000000000000000000, 0.000000000000000000, -0.000000000000000000 ) ) ;
#12316=CARTESIAN_POINT ( 'NONE',  ( 12.00000000000001776, 8.000000000000000000, -6.999999999999999112 ) ) ;
#12317=CIRCLE ( 'NONE', #6440, 1.499999999999999556 ) ;
#12336=DIRECTION ( 'NONE',  ( -1.000000000000000000, -0.000000000000000000, -1.927470528863118802E-16 ) ) ;
#12343=ORIENTED_EDGE ( 'NONE', *, *, #1102, .T. ) ;
#12353=( NAMED_UNIT ( * ) SI_UNIT ( $, .STERADIAN. ) SOLID_ANGLE_UNIT ( ) );
#12381=CARTESIAN_POINT ( 'NONE',  ( 2.999999999999997335, 2.000000000000000000, -7.000000000000001776 ) ) ;
#12393=VECTOR ( 'NONE', #8005, 1000.000000000000000 ) ;
#12397=EDGE_CURVE ( 'NONE', #43, #9336, #687, .T. ) ;
#12403=ORIENTED_EDGE ( 'NONE', *, *, #7812, .T. ) ;
#12432=EDGE_CURVE ( 'NONE', #9336, #8880, #4302, .T. ) ;
#12462=AXIS2_PLACEMENT_3D ( 'NONE', #3184, #4417, #8541 ) ;
#12467=CARTESIAN_POINT ( 'NONE',  ( 10.00000000000001421, 6.000000000000007105, -2.602085213965208275E-15 ) ) ;
#12479=PRODUCT_CONTEXT ( 'NONE', #10114, 'mechanical' ) ;
#12485=ORIENTED_EDGE ( 'NONE', *, *, #13235, .T. ) ;
#12493=LINE ( 'NONE', #2896, #4910 ) ;
#12506=EDGE_CURVE ( 'NONE', #7435, #5535, #5020, .T. ) ;
#12507=CARTESIAN_POINT ( 'NONE',  ( 3.000000000000001776, 2.000000000000000000, 7.000000000000000000 ) ) ;
#12562=ORIENTED_EDGE ( 'NONE', *, *, #10739, .F. ) ;
#12603=DIRECTION ( 'NONE',  ( 0.000000000000000000, 0.000000000000000000, 1.000000000000000000 ) ) ;
#12619=PRODUCT ( 'base-mounting-bracket', 'base-mounting-bracket', '', ( #12479 ) ) ;
#12634=LINE ( 'NONE', #13592, #11716 ) ;
#12639=DIRECTION ( 'NONE',  ( -3.491481338843133355E-15, -1.000000000000000000, 9.085131966639173460E-31 ) ) ;
#12651=LINE ( 'NONE', #10573, #11544 ) ;
#12653=DIRECTION ( 'NONE',  ( 0.000000000000000000, 0.000000000000000000, 1.000000000000000000 ) ) ;
#12657=CARTESIAN_POINT ( 'NONE',  ( 9.250000000000003553, 2.750000000000000888, 10.00000000000000000 ) ) ;
#12660=( GEOMETRIC_REPRESENTATION_CONTEXT ( 3 ) GLOBAL_UNCERTAINTY_ASSIGNED_CONTEXT ( ( #9291 ) ) GLOBAL_UNIT_ASSIGNED_CONTEXT ( ( #11929, #5926, #12353 ) ) REPRESENTATION_CONTEXT ( 'NONE', 'WORKASPACE' ) );
#12663=LINE ( 'NONE', #1146, #4657 ) ;
#12664=EDGE_LOOP ( 'NONE', ( #10484, #9696, #5091, #145 ) ) ;
#12672=LINE ( 'NONE', #72, #9555 ) ;
#12680=PRODUCT_DEFINITION_FORMATION_WITH_SPECIFIED_SOURCE ( 'ANY', '', #12619, .NOT_KNOWN. ) ;
#12688=CARTESIAN_POINT ( 'NONE',  ( 3.000000000000001776, 2.000000000000000000, 10.00000000000000000 ) ) ;
#12706=PLANE ( 'NONE',  #9564 ) ;
#12707=VERTEX_POINT ( 'NONE', #9823 ) ;
#12728=DIRECTION ( 'NONE',  ( 0.000000000000000000, 1.000000000000000000, 0.000000000000000000 ) ) ;
#12763=AXIS2_PLACEMENT_3D ( 'NONE', #7356, #12728, #954 ) ;
#12775=VECTOR ( 'NONE', #7834, 1000.000000000000000 ) ;
#12798=CARTESIAN_POINT ( 'NONE',  ( 11.99999999999999289, -4.861632610112956756E-14, -3.122502256758250798E-15 ) ) ;
#12819=LINE ( 'NONE', #10808, #10631 ) ;
#12834=DIRECTION ( 'NONE',  ( 0.000000000000000000, 1.000000000000000000, 2.891205793294684736E-16 ) ) ;
#12879=ORIENTED_EDGE ( 'NONE', *, *, #11317, .F. ) ;
#12891=FACE_OUTER_BOUND ( 'NONE', #2947, .T. ) ;
#12900=CARTESIAN_POINT ( 'NONE',  ( 9.249999999999996447, -1.734723475976807094E-15, -10.00000000000000178 ) ) ;
#12914=DIRECTION ( 'NONE',  ( 0.000000000000000000, 0.000000000000000000, -1.000000000000000000 ) ) ;
#12918=CARTESIAN_POINT ( 'NONE',  ( 9.250000000000003553, 2.750000000000000888, -10.00000000000000355 ) ) ;
#12938=ADVANCED_FACE ( 'NONE', ( #599 ), #6783, .T. ) ;
#12939=ORIENTED_EDGE ( 'NONE', *, *, #9261, .T. ) ;
#13002=EDGE_LOOP ( 'NONE', ( #4534, #1361, #6137, #3251 ) ) ;
#13010=AXIS2_PLACEMENT_3D ( 'NONE', #1740, #13169, #6973 ) ;
#13025=EDGE_LOOP ( 'NONE', ( #240, #425 ) ) ;
#13061=AXIS2_PLACEMENT_3D ( 'NONE', #9166, #5032, #4196 ) ;
#13078=DIRECTION ( 'NONE',  ( -3.061616997868383141E-16, 0.000000000000000000, -1.000000000000000000 ) ) ;
#13097=EDGE_CURVE ( 'NONE', #11231, #2693, #6253, .T. ) ;
#13100=ORIENTED_EDGE ( 'NONE', *, *, #10073, .T. ) ;
#13124=ORIENTED_EDGE ( 'NONE', *, *, #3526, .T. ) ;
#13136=EDGE_CURVE ( 'NONE', #9925, #9010, #810, .T. ) ;
#13169=DIRECTION ( 'NONE',  ( -1.000000000000000000, 3.469446951953610639E-15, 2.602085213965210149E-16 ) ) ;
#13186=FACE_OUTER_BOUND ( 'NONE', #268, .T. ) ;
#13192=DIRECTION ( 'NONE',  ( -0.000000000000000000, -1.000000000000000000, -0.000000000000000000 ) ) ;
#13194=CARTESIAN_POINT ( 'NONE',  ( 12.00000000000001954, 8.000000000000000000, -6.999999999999999112 ) ) ;
#13221=EDGE_LOOP ( 'NONE', ( #486, #3706, #6344, #5875 ) ) ;
#13235=EDGE_CURVE ( 'NONE', #9925, #4390, #12651, .T. ) ;
#13242=CIRCLE ( 'NONE', #13010, 0.7499999999999997780 ) ;
#13252=CIRCLE ( 'NONE', #7312, 0.7500000000000024425 ) ;
#13269=CARTESIAN_POINT ( 'NONE',  ( 2.720000000000001528, 2.000000000000000000, 4.500000000000000000 ) ) ;
#13306=VECTOR ( 'NONE', #6801, 1000.000000000000000 ) ;
#13315=CARTESIAN_POINT ( 'NONE',  ( 9.250000000000003553, 2.750000000000000888, -10.00000000000000355 ) ) ;
#13317=COLOUR_RGB ( '',0.7921568627450980005, 0.8196078431372548767, 0.9333333333333333481 ) ;
#13355=ORIENTED_EDGE ( 'NONE', *, *, #7731, .T. ) ;
#13366=DIRECTION ( 'NONE',  ( 0.000000000000000000, 0.000000000000000000, 1.000000000000000000 ) ) ;
#13368=VERTEX_POINT ( 'NONE', #6635 ) ;
#13378=FACE_OUTER_BOUND ( 'NONE', #8332, .T. ) ;
#13392=DIRECTION ( 'NONE',  ( -2.312964634635735561E-15, -1.000000000000000000, 0.000000000000000000 ) ) ;
#13394=PLANE ( 'NONE',  #11222 ) ;
#13443=DIRECTION ( 'NONE',  ( -1.000000000000000000, 3.469446951953610639E-15, 2.602085213965210149E-16 ) ) ;
#13448=DIRECTION ( 'NONE',  ( 3.469446951953610639E-15, 1.000000000000000000, 2.891205793294675861E-16 ) ) ;
#13455=LINE ( 'NONE', #1421, #12393 ) ;
#13457=VECTOR ( 'NONE', #9120, 1000.000000000000000 ) ;
#13458=ORIENTED_EDGE ( 'NONE', *, *, #12506, .F. ) ;
#13509=ADVANCED_FACE ( 'NONE', ( #9590 ), #9651, .F. ) ;
#13592=CARTESIAN_POINT ( 'NONE',  ( 9.250000000000001776, 1.999999999999998224, -10.00000000000000355 ) ) ;
#13622=COLOUR_RGB('Dark Blue',0.08,0.2,0.34);
#13623=FILL_AREA_STYLE_COLOUR('',#13622);
#13624=FILL_AREA_STYLE('',(#13623));
#13625=SURFACE_STYLE_FILL_AREA(#13624);
#13626=SURFACE_SIDE_STYLE('',(#13625));
#13627=SURFACE_STYLE_USAGE(.BOTH.,#13626);
#13628=PRESENTATION_STYLE_ASSIGNMENT((#13627));
ENDSEC;
END-ISO-10303-21;
